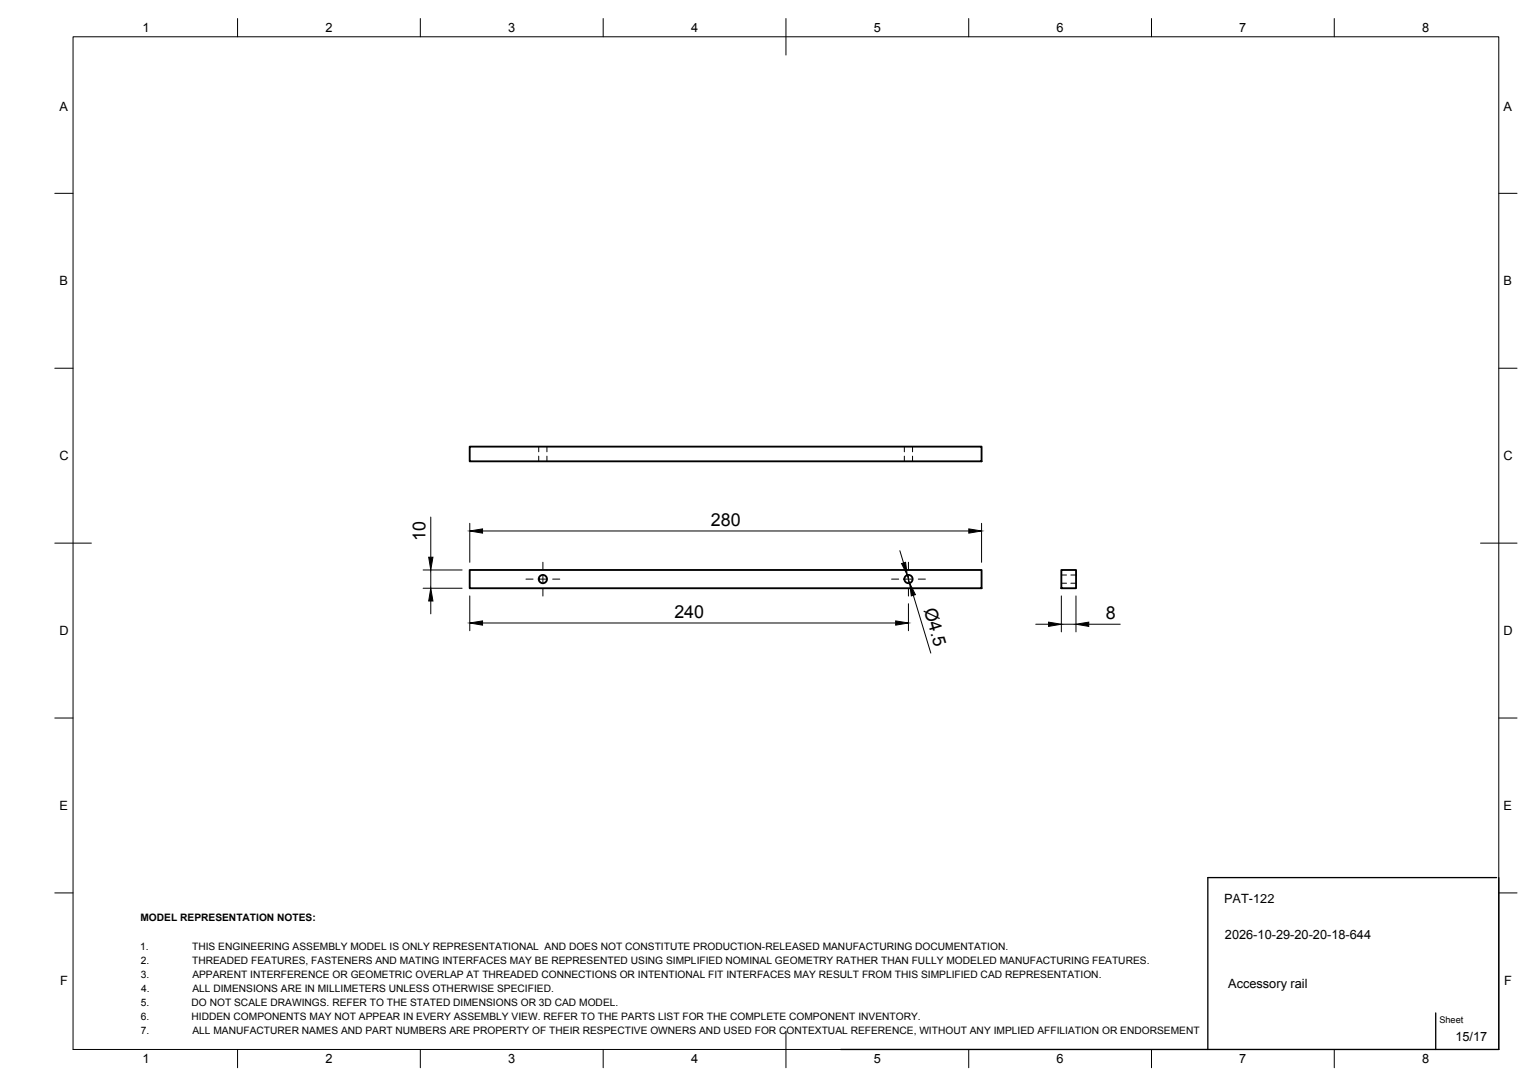
ISO-10303-21;
HEADER;
/* Generated by software containing ST-Developer
 * from STEP Tools, Inc. (www.steptools.com) 
 */

FILE_DESCRIPTION(
/* description */ ('PAT-122'),
/* implementation_level */ '2;1');

FILE_NAME(
/* name */ 'Accessory rail.step',
/* time_stamp */ '2026-10-29T20:20:12-07:00',
/* author */ (''),
/* organization */ (''),
/* preprocessor_version */ 'ST-DEVELOPER v20.2',
/* originating_system */ 'Autodesk Translation Framework v15.17.0.0',
/* authorisation */ '');

FILE_SCHEMA (('AUTOMOTIVE_DESIGN { 1 0 10303 214 3 1 1 }'));
ENDSEC;

DATA;
#10=MECHANICAL_DESIGN_GEOMETRIC_PRESENTATION_REPRESENTATION('',(#503),#10019);
#459=SHAPE_REPRESENTATION_RELATIONSHIP('SRR','None',#10180,#481);
#481=ADVANCED_BREP_SHAPE_REPRESENTATION('',(#525),#10009);
#503=STYLED_ITEM('',(#10334),#525);
#525=MANIFOLD_SOLID_BREP('Body1',#5625);
#579=FACE_BOUND('',#1262,.T.);
#580=FACE_BOUND('',#1263,.T.);
#581=FACE_BOUND('',#1265,.T.);
#582=FACE_BOUND('',#1266,.T.);
#665=PLANE('',#6060);
#666=PLANE('',#6061);
#667=PLANE('',#6062);
#668=PLANE('',#6063);
#669=PLANE('',#6064);
#670=PLANE('',#6065);
#915=FACE_OUTER_BOUND('',#1255,.T.);
#916=FACE_OUTER_BOUND('',#1256,.T.);
#917=FACE_OUTER_BOUND('',#1257,.T.);
#918=FACE_OUTER_BOUND('',#1258,.T.);
#919=FACE_OUTER_BOUND('',#1259,.T.);
#920=FACE_OUTER_BOUND('',#1260,.T.);
#921=FACE_OUTER_BOUND('',#1261,.T.);
#922=FACE_OUTER_BOUND('',#1264,.T.);
#1255=EDGE_LOOP('',(#4237,#4238,#4239,#4240));
#1256=EDGE_LOOP('',(#4241,#4242,#4243,#4244));
#1257=EDGE_LOOP('',(#4245,#4246,#4247,#4248));
#1258=EDGE_LOOP('',(#4249,#4250,#4251,#4252));
#1259=EDGE_LOOP('',(#4253,#4254,#4255,#4256));
#1260=EDGE_LOOP('',(#4257,#4258,#4259,#4260));
#1261=EDGE_LOOP('',(#4261,#4262,#4263,#4264));
#1262=EDGE_LOOP('',(#4265));
#1263=EDGE_LOOP('',(#4266));
#1264=EDGE_LOOP('',(#4267,#4268,#4269,#4270));
#1265=EDGE_LOOP('',(#4271));
#1266=EDGE_LOOP('',(#4272));
#1605=LINE('',#8476,#2149);
#1606=LINE('',#8482,#2150);
#1607=LINE('',#8487,#2151);
#1608=LINE('',#8489,#2152);
#1609=LINE('',#8491,#2153);
#1610=LINE('',#8492,#2154);
#1611=LINE('',#8495,#2155);
#1612=LINE('',#8497,#2156);
#1613=LINE('',#8498,#2157);
#1614=LINE('',#8501,#2158);
#1615=LINE('',#8503,#2159);
#1616=LINE('',#8504,#2160);
#1617=LINE('',#8506,#2161);
#1618=LINE('',#8507,#2162);
#2149=VECTOR('',#6892,0.225);
#2150=VECTOR('',#6899,0.225);
#2151=VECTOR('',#6904,1.);
#2152=VECTOR('',#6905,1.);
#2153=VECTOR('',#6906,1.);
#2154=VECTOR('',#6907,1.);
#2155=VECTOR('',#6910,1.);
#2156=VECTOR('',#6911,1.);
#2157=VECTOR('',#6912,1.);
#2158=VECTOR('',#6915,1.);
#2159=VECTOR('',#6916,1.);
#2160=VECTOR('',#6917,1.);
#2161=VECTOR('',#6920,1.);
#2162=VECTOR('',#6921,1.);
#2643=CIRCLE('',#6055,0.225);
#2644=CIRCLE('',#6056,0.225);
#2645=CIRCLE('',#6058,0.225);
#2646=CIRCLE('',#6059,0.225);
#2829=VERTEX_POINT('',#8473);
#2830=VERTEX_POINT('',#8475);
#2831=VERTEX_POINT('',#8479);
#2832=VERTEX_POINT('',#8481);
#2833=VERTEX_POINT('',#8485);
#2834=VERTEX_POINT('',#8486);
#2835=VERTEX_POINT('',#8488);
#2836=VERTEX_POINT('',#8490);
#2837=VERTEX_POINT('',#8494);
#2838=VERTEX_POINT('',#8496);
#2839=VERTEX_POINT('',#8500);
#2840=VERTEX_POINT('',#8502);
#3353=EDGE_CURVE('',#2829,#2829,#2643,.T.);
#3354=EDGE_CURVE('',#2829,#2830,#1605,.T.);
#3355=EDGE_CURVE('',#2830,#2830,#2644,.T.);
#3356=EDGE_CURVE('',#2831,#2831,#2645,.T.);
#3357=EDGE_CURVE('',#2831,#2832,#1606,.T.);
#3358=EDGE_CURVE('',#2832,#2832,#2646,.T.);
#3359=EDGE_CURVE('',#2833,#2834,#1607,.T.);
#3360=EDGE_CURVE('',#2834,#2835,#1608,.T.);
#3361=EDGE_CURVE('',#2836,#2835,#1609,.T.);
#3362=EDGE_CURVE('',#2833,#2836,#1610,.T.);
#3363=EDGE_CURVE('',#2837,#2833,#1611,.T.);
#3364=EDGE_CURVE('',#2838,#2836,#1612,.T.);
#3365=EDGE_CURVE('',#2837,#2838,#1613,.T.);
#3366=EDGE_CURVE('',#2839,#2837,#1614,.T.);
#3367=EDGE_CURVE('',#2840,#2838,#1615,.T.);
#3368=EDGE_CURVE('',#2839,#2840,#1616,.T.);
#3369=EDGE_CURVE('',#2834,#2839,#1617,.T.);
#3370=EDGE_CURVE('',#2835,#2840,#1618,.T.);
#4237=ORIENTED_EDGE('',*,*,#3353,.F.);
#4238=ORIENTED_EDGE('',*,*,#3354,.T.);
#4239=ORIENTED_EDGE('',*,*,#3355,.F.);
#4240=ORIENTED_EDGE('',*,*,#3354,.F.);
#4241=ORIENTED_EDGE('',*,*,#3356,.F.);
#4242=ORIENTED_EDGE('',*,*,#3357,.T.);
#4243=ORIENTED_EDGE('',*,*,#3358,.F.);
#4244=ORIENTED_EDGE('',*,*,#3357,.F.);
#4245=ORIENTED_EDGE('',*,*,#3359,.T.);
#4246=ORIENTED_EDGE('',*,*,#3360,.T.);
#4247=ORIENTED_EDGE('',*,*,#3361,.F.);
#4248=ORIENTED_EDGE('',*,*,#3362,.F.);
#4249=ORIENTED_EDGE('',*,*,#3363,.T.);
#4250=ORIENTED_EDGE('',*,*,#3362,.T.);
#4251=ORIENTED_EDGE('',*,*,#3364,.F.);
#4252=ORIENTED_EDGE('',*,*,#3365,.F.);
#4253=ORIENTED_EDGE('',*,*,#3366,.T.);
#4254=ORIENTED_EDGE('',*,*,#3365,.T.);
#4255=ORIENTED_EDGE('',*,*,#3367,.F.);
#4256=ORIENTED_EDGE('',*,*,#3368,.F.);
#4257=ORIENTED_EDGE('',*,*,#3369,.T.);
#4258=ORIENTED_EDGE('',*,*,#3368,.T.);
#4259=ORIENTED_EDGE('',*,*,#3370,.F.);
#4260=ORIENTED_EDGE('',*,*,#3360,.F.);
#4261=ORIENTED_EDGE('',*,*,#3370,.T.);
#4262=ORIENTED_EDGE('',*,*,#3367,.T.);
#4263=ORIENTED_EDGE('',*,*,#3364,.T.);
#4264=ORIENTED_EDGE('',*,*,#3361,.T.);
#4265=ORIENTED_EDGE('',*,*,#3355,.T.);
#4266=ORIENTED_EDGE('',*,*,#3358,.T.);
#4267=ORIENTED_EDGE('',*,*,#3369,.F.);
#4268=ORIENTED_EDGE('',*,*,#3359,.F.);
#4269=ORIENTED_EDGE('',*,*,#3363,.F.);
#4270=ORIENTED_EDGE('',*,*,#3366,.F.);
#4271=ORIENTED_EDGE('',*,*,#3353,.T.);
#4272=ORIENTED_EDGE('',*,*,#3356,.T.);
#5295=CYLINDRICAL_SURFACE('',#6054,0.225);
#5296=CYLINDRICAL_SURFACE('',#6057,0.225);
#5411=ADVANCED_FACE('',(#915),#5295,.F.);
#5412=ADVANCED_FACE('',(#916),#5296,.F.);
#5413=ADVANCED_FACE('',(#917),#665,.T.);
#5414=ADVANCED_FACE('',(#918),#666,.T.);
#5415=ADVANCED_FACE('',(#919),#667,.T.);
#5416=ADVANCED_FACE('',(#920),#668,.T.);
#5417=ADVANCED_FACE('',(#921,#579,#580),#669,.T.);
#5418=ADVANCED_FACE('',(#922,#581,#582),#670,.F.);
#5625=CLOSED_SHELL('',(#5411,#5412,#5413,#5414,#5415,#5416,#5417,#5418));
#6053=AXIS2_PLACEMENT_3D('',#8471,#6886,#6887);
#6054=AXIS2_PLACEMENT_3D('',#8472,#6888,#6889);
#6055=AXIS2_PLACEMENT_3D('',#8474,#6890,#6891);
#6056=AXIS2_PLACEMENT_3D('',#8477,#6893,#6894);
#6057=AXIS2_PLACEMENT_3D('',#8478,#6895,#6896);
#6058=AXIS2_PLACEMENT_3D('',#8480,#6897,#6898);
#6059=AXIS2_PLACEMENT_3D('',#8483,#6900,#6901);
#6060=AXIS2_PLACEMENT_3D('',#8484,#6902,#6903);
#6061=AXIS2_PLACEMENT_3D('',#8493,#6908,#6909);
#6062=AXIS2_PLACEMENT_3D('',#8499,#6913,#6914);
#6063=AXIS2_PLACEMENT_3D('',#8505,#6918,#6919);
#6064=AXIS2_PLACEMENT_3D('',#8508,#6922,#6923);
#6065=AXIS2_PLACEMENT_3D('',#8509,#6924,#6925);
#6886=DIRECTION('axis',(0.,0.,1.));
#6887=DIRECTION('refdir',(1.,0.,0.));
#6888=DIRECTION('center_axis',(0.,0.,1.));
#6889=DIRECTION('ref_axis',(1.,0.,0.));
#6890=DIRECTION('center_axis',(0.,0.,1.));
#6891=DIRECTION('ref_axis',(1.,0.,0.));
#6892=DIRECTION('',(0.,0.,1.));
#6893=DIRECTION('center_axis',(0.,0.,-1.));
#6894=DIRECTION('ref_axis',(1.,0.,0.));
#6895=DIRECTION('center_axis',(0.,0.,1.));
#6896=DIRECTION('ref_axis',(1.,0.,0.));
#6897=DIRECTION('center_axis',(0.,0.,1.));
#6898=DIRECTION('ref_axis',(1.,0.,0.));
#6899=DIRECTION('',(0.,0.,1.));
#6900=DIRECTION('center_axis',(0.,0.,-1.));
#6901=DIRECTION('ref_axis',(1.,0.,0.));
#6902=DIRECTION('center_axis',(0.,1.,0.));
#6903=DIRECTION('ref_axis',(-1.,0.,0.));
#6904=DIRECTION('',(-1.,0.,0.));
#6905=DIRECTION('',(0.,0.,1.));
#6906=DIRECTION('',(-1.,0.,0.));
#6907=DIRECTION('',(0.,0.,1.));
#6908=DIRECTION('center_axis',(1.,0.,0.));
#6909=DIRECTION('ref_axis',(0.,1.,0.));
#6910=DIRECTION('',(0.,1.,0.));
#6911=DIRECTION('',(0.,1.,0.));
#6912=DIRECTION('',(0.,0.,1.));
#6913=DIRECTION('center_axis',(0.,-1.,0.));
#6914=DIRECTION('ref_axis',(1.,0.,0.));
#6915=DIRECTION('',(1.,0.,0.));
#6916=DIRECTION('',(1.,0.,0.));
#6917=DIRECTION('',(0.,0.,1.));
#6918=DIRECTION('center_axis',(-1.,0.,0.));
#6919=DIRECTION('ref_axis',(0.,-1.,0.));
#6920=DIRECTION('',(0.,-1.,0.));
#6921=DIRECTION('',(0.,-1.,0.));
#6922=DIRECTION('center_axis',(0.,0.,1.));
#6923=DIRECTION('ref_axis',(1.,0.,0.));
#6924=DIRECTION('center_axis',(0.,0.,1.));
#6925=DIRECTION('ref_axis',(1.,0.,0.));
#8471=CARTESIAN_POINT('',(0.,0.,0.));
#8472=CARTESIAN_POINT('Origin',(-10.,22.5,39.7));
#8473=CARTESIAN_POINT('',(-10.225,22.5,39.8));
#8474=CARTESIAN_POINT('Origin',(-10.,22.5,39.8));
#8475=CARTESIAN_POINT('',(-10.225,22.5,40.6));
#8476=CARTESIAN_POINT('',(-10.225,22.5,39.7));
#8477=CARTESIAN_POINT('Origin',(-10.,22.5,40.6));
#8478=CARTESIAN_POINT('Origin',(10.,22.5,39.7));
#8479=CARTESIAN_POINT('',(9.775,22.5,39.8));
#8480=CARTESIAN_POINT('Origin',(10.,22.5,39.8));
#8481=CARTESIAN_POINT('',(9.775,22.5,40.6));
#8482=CARTESIAN_POINT('',(9.775,22.5,39.7));
#8483=CARTESIAN_POINT('Origin',(10.,22.5,40.6));
#8484=CARTESIAN_POINT('Origin',(14.,23.,39.8));
#8485=CARTESIAN_POINT('',(14.,23.,39.8));
#8486=CARTESIAN_POINT('',(-14.,23.,39.8));
#8487=CARTESIAN_POINT('',(14.,23.,39.8));
#8488=CARTESIAN_POINT('',(-14.,23.,40.6));
#8489=CARTESIAN_POINT('',(-14.,23.,39.8));
#8490=CARTESIAN_POINT('',(14.,23.,40.6));
#8491=CARTESIAN_POINT('',(14.,23.,40.6));
#8492=CARTESIAN_POINT('',(14.,23.,39.8));
#8493=CARTESIAN_POINT('Origin',(14.,22.,39.8));
#8494=CARTESIAN_POINT('',(14.,22.,39.8));
#8495=CARTESIAN_POINT('',(14.,22.,39.8));
#8496=CARTESIAN_POINT('',(14.,22.,40.6));
#8497=CARTESIAN_POINT('',(14.,22.,40.6));
#8498=CARTESIAN_POINT('',(14.,22.,39.8));
#8499=CARTESIAN_POINT('Origin',(-14.,22.,39.8));
#8500=CARTESIAN_POINT('',(-14.,22.,39.8));
#8501=CARTESIAN_POINT('',(-14.,22.,39.8));
#8502=CARTESIAN_POINT('',(-14.,22.,40.6));
#8503=CARTESIAN_POINT('',(-14.,22.,40.6));
#8504=CARTESIAN_POINT('',(-14.,22.,39.8));
#8505=CARTESIAN_POINT('Origin',(-14.,23.,39.8));
#8506=CARTESIAN_POINT('',(-14.,23.,39.8));
#8507=CARTESIAN_POINT('',(-14.,23.,40.6));
#8508=CARTESIAN_POINT('Origin',(0.,22.5,40.6));
#8509=CARTESIAN_POINT('Origin',(0.,22.5,39.8));
#9985=UNCERTAINTY_MEASURE_WITH_UNIT(LENGTH_MEASURE(0.001),#10020,
'DISTANCE_ACCURACY_VALUE',
'Maximum model space distance between geometric entities at asserted c
onnectivities');
#9995=UNCERTAINTY_MEASURE_WITH_UNIT(LENGTH_MEASURE(0.001),#10020,
'DISTANCE_ACCURACY_VALUE',
'Maximum model space distance between geometric entities at asserted c
onnectivities');
#10009=(
GEOMETRIC_REPRESENTATION_CONTEXT(3)
GLOBAL_UNCERTAINTY_ASSIGNED_CONTEXT((#9985))
GLOBAL_UNIT_ASSIGNED_CONTEXT((#10020,#10022,#10023))
REPRESENTATION_CONTEXT('','3D')
);
#10019=(
GEOMETRIC_REPRESENTATION_CONTEXT(3)
GLOBAL_UNCERTAINTY_ASSIGNED_CONTEXT((#9995))
GLOBAL_UNIT_ASSIGNED_CONTEXT((#10020,#10022,#10023))
REPRESENTATION_CONTEXT('','3D')
);
#10020=(
LENGTH_UNIT()
NAMED_UNIT(*)
SI_UNIT(.CENTI.,.METRE.)
);
#10022=(
NAMED_UNIT(*)
PLANE_ANGLE_UNIT()
SI_UNIT($,.RADIAN.)
);
#10023=(
NAMED_UNIT(*)
SI_UNIT($,.STERADIAN.)
SOLID_ANGLE_UNIT()
);
#10037=SHAPE_DEFINITION_REPRESENTATION(#10060,#10180);
#10060=PRODUCT_DEFINITION_SHAPE('',$,#10204);
#10180=SHAPE_REPRESENTATION('',(#6053),#10009);
#10190=PRODUCT_DEFINITION_CONTEXT('part definition',#10261,'design');
#10204=PRODUCT_DEFINITION('Accessory rail','Accessory rail',
#10227,#10190);
#10227=PRODUCT_DEFINITION_FORMATION('',$,#10276);
#10261=APPLICATION_CONTEXT(
'Core Data for Automotive Mechanical Design Process');
#10262=PRODUCT_CONTEXT('part definition',#10261,'mechanical');
#10276=PRODUCT('Accessory rail','Accessory rail',
'Accessory rail',(#10262));
#10328=COLOUR_RGB('Light Blue',0.38,0.62,0.78);
#10329=FILL_AREA_STYLE_COLOUR('',#10328);
#10330=FILL_AREA_STYLE('',(#10329));
#10331=SURFACE_STYLE_FILL_AREA(#10330);
#10332=SURFACE_SIDE_STYLE('',(#10331));
#10333=SURFACE_STYLE_USAGE(.BOTH.,#10332);
#10334=PRESENTATION_STYLE_ASSIGNMENT((#10333));
ENDSEC;
END-ISO-10303-21;
